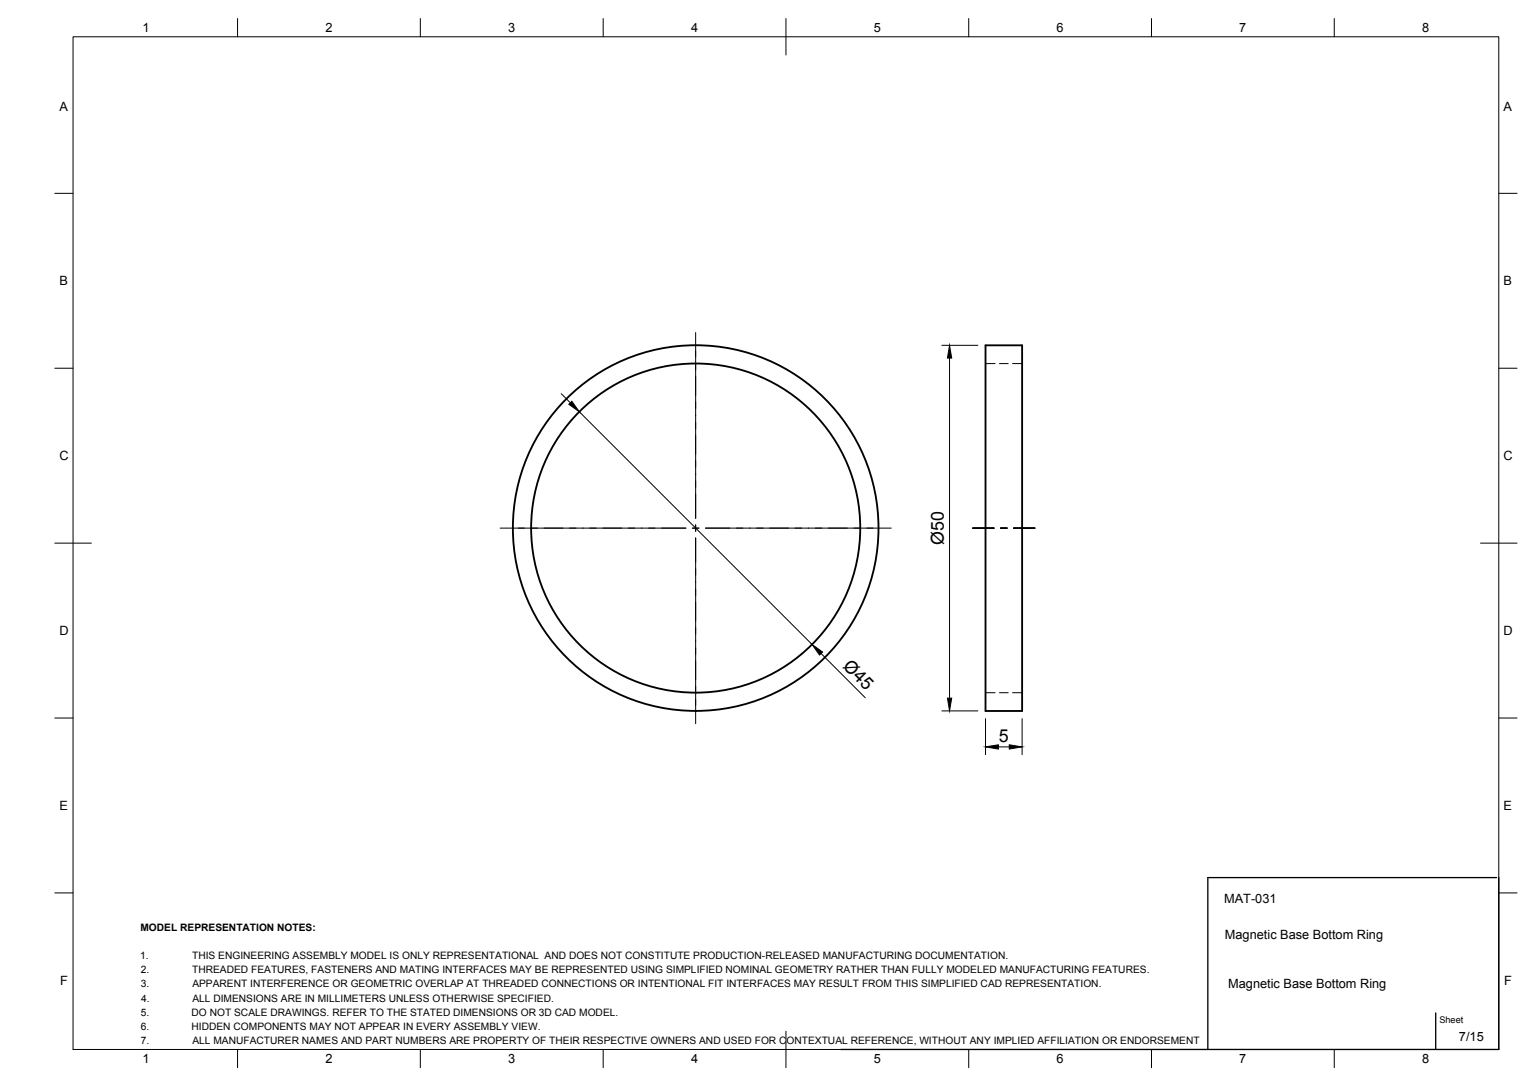
ISO-10303-21;
HEADER;
/* Generated by software containing ST-Developer
 * from STEP Tools, Inc. (www.steptools.com) 
 */

FILE_DESCRIPTION(
/* description */ ('STEP AP214'),
/* implementation_level */ '2;1');

FILE_NAME(
/* name */ 'Magnetic Base Bottom Ring.step',
/* time_stamp */ '2026-11-14T06:58:01-08:00',
/* author */ (''),
/* organization */ (''),
/* preprocessor_version */ 'ST-DEVELOPER v20.2',
/* originating_system */ 'Autodesk Translation Framework v15.17.0.0',
/* authorisation */ '');

FILE_SCHEMA (('AUTOMOTIVE_DESIGN { 1 0 10303 214 3 1 1 }'));
ENDSEC;

DATA;
#10=MECHANICAL_DESIGN_GEOMETRIC_PRESENTATION_REPRESENTATION('',(#1150),#38635);
#870=FACE_BOUND('',#2805,.T.);
#871=FACE_BOUND('',#2807,.T.);
#1116=SHAPE_REPRESENTATION_RELATIONSHIP('SRR','None',#38689,#1130);
#1130=ADVANCED_BREP_SHAPE_REPRESENTATION('',(#1176),#38625);
#1150=STYLED_ITEM('',(#38766),#1176);
#1176=MANIFOLD_SOLID_BREP('Body1',#17616);
#1248=PLANE('',#18019);
#1249=PLANE('',#18020);
#1788=FACE_OUTER_BOUND('',#2802,.T.);
#1789=FACE_OUTER_BOUND('',#2803,.T.);
#1790=FACE_OUTER_BOUND('',#2804,.T.);
#1791=FACE_OUTER_BOUND('',#2806,.T.);
#2802=EDGE_LOOP('',(#11637,#11638,#11639,#11640));
#2803=EDGE_LOOP('',(#11641,#11642,#11643,#11644));
#2804=EDGE_LOOP('',(#11645));
#2805=EDGE_LOOP('',(#11646));
#2806=EDGE_LOOP('',(#11647));
#2807=EDGE_LOOP('',(#11648));
#3875=LINE('',#29907,#4819);
#3876=LINE('',#29913,#4820);
#4819=VECTOR('',#20376,22.5);
#4820=VECTOR('',#20383,25.);
#5663=CIRCLE('',#18014,22.5);
#5664=CIRCLE('',#18015,22.5);
#5665=CIRCLE('',#18017,25.);
#5666=CIRCLE('',#18018,25.);
#6753=VERTEX_POINT('',#29904);
#6754=VERTEX_POINT('',#29906);
#6755=VERTEX_POINT('',#29910);
#6756=VERTEX_POINT('',#29912);
#8605=EDGE_CURVE('',#6753,#6753,#5663,.T.);
#8606=EDGE_CURVE('',#6753,#6754,#3875,.T.);
#8607=EDGE_CURVE('',#6754,#6754,#5664,.T.);
#8608=EDGE_CURVE('',#6755,#6755,#5665,.T.);
#8609=EDGE_CURVE('',#6755,#6756,#3876,.T.);
#8610=EDGE_CURVE('',#6756,#6756,#5666,.T.);
#11637=ORIENTED_EDGE('',*,*,#8605,.T.);
#11638=ORIENTED_EDGE('',*,*,#8606,.T.);
#11639=ORIENTED_EDGE('',*,*,#8607,.F.);
#11640=ORIENTED_EDGE('',*,*,#8606,.F.);
#11641=ORIENTED_EDGE('',*,*,#8608,.T.);
#11642=ORIENTED_EDGE('',*,*,#8609,.T.);
#11643=ORIENTED_EDGE('',*,*,#8610,.F.);
#11644=ORIENTED_EDGE('',*,*,#8609,.F.);
#11645=ORIENTED_EDGE('',*,*,#8610,.T.);
#11646=ORIENTED_EDGE('',*,*,#8605,.F.);
#11647=ORIENTED_EDGE('',*,*,#8608,.F.);
#11648=ORIENTED_EDGE('',*,*,#8607,.T.);
#16325=CYLINDRICAL_SURFACE('',#18013,22.5);
#16326=CYLINDRICAL_SURFACE('',#18016,25.);
#16747=ADVANCED_FACE('',(#1788),#16325,.F.);
#16748=ADVANCED_FACE('',(#1789),#16326,.T.);
#16749=ADVANCED_FACE('',(#1790,#870),#1248,.T.);
#16750=ADVANCED_FACE('',(#1791,#871),#1249,.F.);
#17616=CLOSED_SHELL('',(#16747,#16748,#16749,#16750));
#18012=AXIS2_PLACEMENT_3D('',#29902,#20370,#20371);
#18013=AXIS2_PLACEMENT_3D('',#29903,#20372,#20373);
#18014=AXIS2_PLACEMENT_3D('',#29905,#20374,#20375);
#18015=AXIS2_PLACEMENT_3D('',#29908,#20377,#20378);
#18016=AXIS2_PLACEMENT_3D('',#29909,#20379,#20380);
#18017=AXIS2_PLACEMENT_3D('',#29911,#20381,#20382);
#18018=AXIS2_PLACEMENT_3D('',#29914,#20384,#20385);
#18019=AXIS2_PLACEMENT_3D('',#29915,#20386,#20387);
#18020=AXIS2_PLACEMENT_3D('',#29916,#20388,#20389);
#20370=DIRECTION('axis',(0.,0.,1.));
#20371=DIRECTION('refdir',(1.,0.,0.));
#20372=DIRECTION('center_axis',(0.,-1.,0.));
#20373=DIRECTION('ref_axis',(0.,0.,-1.));
#20374=DIRECTION('center_axis',(0.,1.,0.));
#20375=DIRECTION('ref_axis',(0.,0.,1.));
#20376=DIRECTION('',(0.,-1.,0.));
#20377=DIRECTION('center_axis',(0.,1.,0.));
#20378=DIRECTION('ref_axis',(0.,0.,1.));
#20379=DIRECTION('center_axis',(0.,-1.,0.));
#20380=DIRECTION('ref_axis',(0.,0.,-1.));
#20381=DIRECTION('center_axis',(0.,1.,0.));
#20382=DIRECTION('ref_axis',(0.,0.,1.));
#20383=DIRECTION('',(0.,1.,0.));
#20384=DIRECTION('center_axis',(0.,1.,0.));
#20385=DIRECTION('ref_axis',(0.,0.,1.));
#20386=DIRECTION('center_axis',(0.,1.,0.));
#20387=DIRECTION('ref_axis',(0.,0.,1.));
#20388=DIRECTION('center_axis',(0.,1.,0.));
#20389=DIRECTION('ref_axis',(0.,0.,1.));
#29902=CARTESIAN_POINT('',(0.,0.,0.));
#29903=CARTESIAN_POINT('Origin',(0.,5.,0.));
#29904=CARTESIAN_POINT('',(-2.75545529808155E-15,5.,22.5));
#29905=CARTESIAN_POINT('Origin',(0.,5.,0.));
#29906=CARTESIAN_POINT('',(-2.75545529808155E-15,0.,22.5));
#29907=CARTESIAN_POINT('',(-2.75545529808155E-15,5.,22.5));
#29908=CARTESIAN_POINT('Origin',(0.,0.,0.));
#29909=CARTESIAN_POINT('Origin',(0.,5.,0.));
#29910=CARTESIAN_POINT('',(-3.06161699786838E-15,0.,25.));
#29911=CARTESIAN_POINT('Origin',(0.,0.,0.));
#29912=CARTESIAN_POINT('',(-3.06161699786838E-15,5.,25.));
#29913=CARTESIAN_POINT('',(-3.06161699786838E-15,5.,25.));
#29914=CARTESIAN_POINT('Origin',(0.,5.,0.));
#29915=CARTESIAN_POINT('Origin',(0.,5.,0.));
#29916=CARTESIAN_POINT('Origin',(0.,0.,0.));
#38609=UNCERTAINTY_MEASURE_WITH_UNIT(LENGTH_MEASURE(0.01),#38636,
'DISTANCE_ACCURACY_VALUE',
'Maximum model space distance between geometric entities at asserted c
onnectivities');
#38619=UNCERTAINTY_MEASURE_WITH_UNIT(LENGTH_MEASURE(0.01),#38636,
'DISTANCE_ACCURACY_VALUE',
'Maximum model space distance between geometric entities at asserted c
onnectivities');
#38625=(
GEOMETRIC_REPRESENTATION_CONTEXT(3)
GLOBAL_UNCERTAINTY_ASSIGNED_CONTEXT((#38609))
GLOBAL_UNIT_ASSIGNED_CONTEXT((#38636,#38638,#38639))
REPRESENTATION_CONTEXT('','3D')
);
#38635=(
GEOMETRIC_REPRESENTATION_CONTEXT(3)
GLOBAL_UNCERTAINTY_ASSIGNED_CONTEXT((#38619))
GLOBAL_UNIT_ASSIGNED_CONTEXT((#38636,#38638,#38639))
REPRESENTATION_CONTEXT('','3D')
);
#38636=(
LENGTH_UNIT()
NAMED_UNIT(*)
SI_UNIT(.MILLI.,.METRE.)
);
#38638=(
NAMED_UNIT(*)
PLANE_ANGLE_UNIT()
SI_UNIT($,.RADIAN.)
);
#38639=(
NAMED_UNIT(*)
SI_UNIT($,.STERADIAN.)
SOLID_ANGLE_UNIT()
);
#38645=SHAPE_DEFINITION_REPRESENTATION(#38660,#38689);
#38660=PRODUCT_DEFINITION_SHAPE('',$,#38705);
#38689=SHAPE_REPRESENTATION('',(#18012),#38625);
#38699=PRODUCT_DEFINITION_CONTEXT('part definition',#38746,'design');
#38705=PRODUCT_DEFINITION('Magnetic Base Bottom Ring',
'Magnetic Base Bottom Ring',#38720,#38699);
#38720=PRODUCT_DEFINITION_FORMATION('',$,#38753);
#38746=APPLICATION_CONTEXT(
'Core Data for Automotive Mechanical Design Process');
#38747=PRODUCT_CONTEXT('part definition',#38746,'mechanical');
#38753=PRODUCT('Magnetic Base Bottom Ring','Magnetic Base Bottom Ring',
$,(#38747));
#38766=PRESENTATION_STYLE_ASSIGNMENT((#38773));
#38773=SURFACE_STYLE_USAGE(.BOTH.,#38780);
#38780=SURFACE_SIDE_STYLE('',(#38787));
#38787=SURFACE_STYLE_FILL_AREA(#38794);
#38794=FILL_AREA_STYLE('Opaque(61,176,222)',(#38801));
#38801=FILL_AREA_STYLE_COLOUR('Opaque(61,176,222)',#38808);
#38808=COLOUR_RGB('Opaque(61,176,222)',0.23921568627451,0.690196078431373,
0.870588235294118);
ENDSEC;
END-ISO-10303-21;
